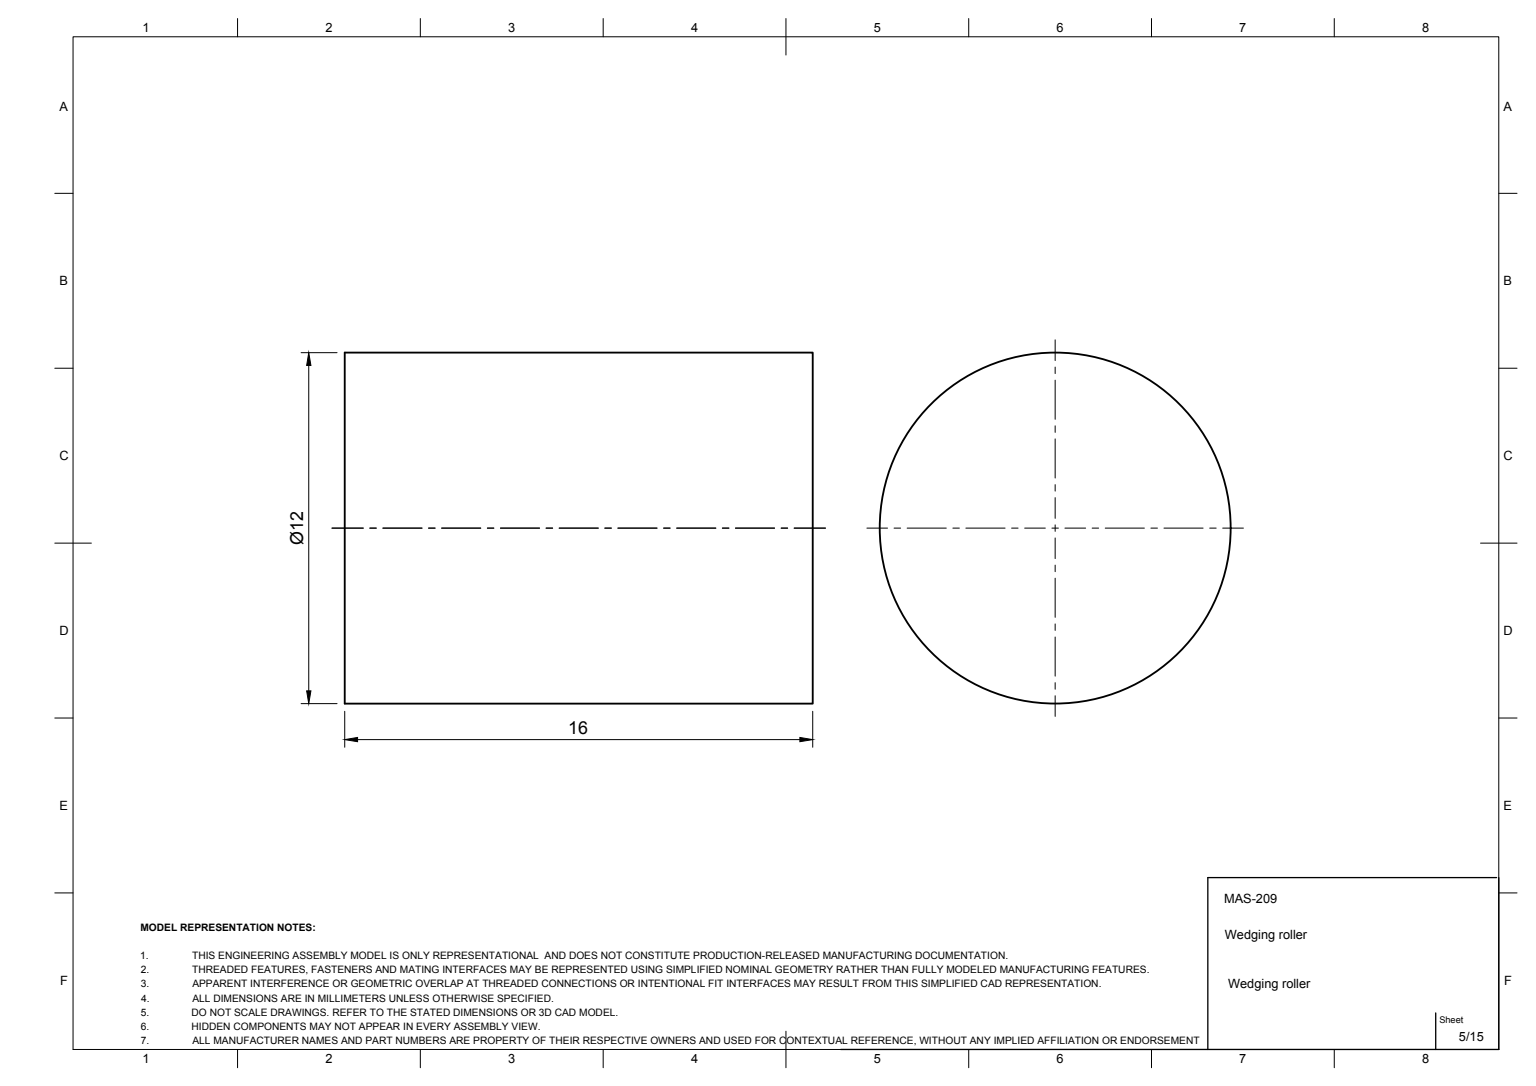
ISO-10303-21;
HEADER;
/* Generated by software containing ST-Developer
 * from STEP Tools, Inc. (www.steptools.com) 
 */

FILE_DESCRIPTION(
/* description */ ('Independent bearing-supported roller-ramp one-way clutch. Six logarit
hmic ramps with plain solid rollers, sprung guided plungers, native Co
il variants, removable shared keepers, rounded parallel key, shaft wit
h complete retaining lips, bronze journal/thrust support and bolted co
vers. Native rotor, roller planar/spin and plunger joints permit manua
l geometric engaged/released inspection. Automatic frictional torque s
witching/contact dynamics are not simulated; no capacity, hardness, fi
t, lubrication, speed, force or life rating. External input driver/cou
pling/anchors outside assembly.'),
/* implementation_level */ '2;1');

FILE_NAME(
/* name */ 'Wedging roller.step',
/* time_stamp */ '2026-11-08T07:04:38-08:00',
/* author */ (''),
/* organization */ (''),
/* preprocessor_version */ 'ST-DEVELOPER v20.2',
/* originating_system */ 'Autodesk Translation Framework v15.17.0.0',
/* authorisation */ '');

FILE_SCHEMA (('AUTOMOTIVE_DESIGN { 1 0 10303 214 3 1 1 }'));
ENDSEC;

DATA;
#10=MECHANICAL_DESIGN_GEOMETRIC_PRESENTATION_REPRESENTATION('',(#304),#99526);
#272=SHAPE_REPRESENTATION_RELATIONSHIP('SRR','None',#99629,#288);
#288=ADVANCED_BREP_SHAPE_REPRESENTATION('',(#320),#99514);
#304=STYLED_ITEM('',(#99718),#320);
#320=MANIFOLD_SOLID_BREP('Body1',#18274);
#565=PLANE('',#19493);
#566=PLANE('',#19494);
#1521=FACE_OUTER_BOUND('',#2580,.T.);
#1522=FACE_OUTER_BOUND('',#2581,.T.);
#1523=FACE_OUTER_BOUND('',#2582,.T.);
#2580=EDGE_LOOP('',(#15846,#15847,#15848,#15849));
#2581=EDGE_LOOP('',(#15850));
#2582=EDGE_LOOP('',(#15851));
#3020=CIRCLE('',#19491,6.);
#3021=CIRCLE('',#19492,6.);
#5399=LINE('',#94662,#6303);
#6303=VECTOR('',#22626,6.);
#8035=VERTEX_POINT('',#94659);
#8036=VERTEX_POINT('',#94661);
#10675=EDGE_CURVE('',#8035,#8035,#3020,.T.);
#10676=EDGE_CURVE('',#8035,#8036,#5399,.T.);
#10677=EDGE_CURVE('',#8036,#8036,#3021,.T.);
#15846=ORIENTED_EDGE('',*,*,#10675,.F.);
#15847=ORIENTED_EDGE('',*,*,#10676,.T.);
#15848=ORIENTED_EDGE('',*,*,#10677,.T.);
#15849=ORIENTED_EDGE('',*,*,#10676,.F.);
#15850=ORIENTED_EDGE('',*,*,#10675,.T.);
#15851=ORIENTED_EDGE('',*,*,#10677,.F.);
#17185=CYLINDRICAL_SURFACE('',#19490,6.);
#18119=ADVANCED_FACE('',(#1521),#17185,.T.);
#18120=ADVANCED_FACE('',(#1522),#565,.T.);
#18121=ADVANCED_FACE('',(#1523),#566,.F.);
#18274=CLOSED_SHELL('',(#18119,#18120,#18121));
#19489=AXIS2_PLACEMENT_3D('',#94657,#22620,#22621);
#19490=AXIS2_PLACEMENT_3D('',#94658,#22622,#22623);
#19491=AXIS2_PLACEMENT_3D('',#94660,#22624,#22625);
#19492=AXIS2_PLACEMENT_3D('',#94663,#22627,#22628);
#19493=AXIS2_PLACEMENT_3D('',#94664,#22629,#22630);
#19494=AXIS2_PLACEMENT_3D('',#94665,#22631,#22632);
#22620=DIRECTION('axis',(0.,0.,1.));
#22621=DIRECTION('refdir',(1.,0.,0.));
#22622=DIRECTION('center_axis',(0.,0.,1.));
#22623=DIRECTION('ref_axis',(1.,0.,0.));
#22624=DIRECTION('center_axis',(0.,0.,1.));
#22625=DIRECTION('ref_axis',(1.,0.,0.));
#22626=DIRECTION('',(0.,0.,-1.));
#22627=DIRECTION('center_axis',(0.,0.,1.));
#22628=DIRECTION('ref_axis',(1.,0.,0.));
#22629=DIRECTION('center_axis',(0.,0.,1.));
#22630=DIRECTION('ref_axis',(1.,0.,0.));
#22631=DIRECTION('center_axis',(0.,0.,1.));
#22632=DIRECTION('ref_axis',(1.,0.,0.));
#94657=CARTESIAN_POINT('',(0.,0.,0.));
#94658=CARTESIAN_POINT('Origin',(0.,0.,0.));
#94659=CARTESIAN_POINT('',(-6.,-7.34788079488412E-16,16.));
#94660=CARTESIAN_POINT('Origin',(0.,0.,16.));
#94661=CARTESIAN_POINT('',(-6.,-7.34788079488412E-16,0.));
#94662=CARTESIAN_POINT('',(-6.,-7.34788079488412E-16,0.));
#94663=CARTESIAN_POINT('Origin',(0.,0.,0.));
#94664=CARTESIAN_POINT('Origin',(0.,0.,16.));
#94665=CARTESIAN_POINT('Origin',(0.,0.,0.));
#99496=UNCERTAINTY_MEASURE_WITH_UNIT(LENGTH_MEASURE(0.01),#99527,
'DISTANCE_ACCURACY_VALUE',
'Maximum model space distance between geometric entities at asserted c
onnectivities');
#99508=UNCERTAINTY_MEASURE_WITH_UNIT(LENGTH_MEASURE(0.01),#99527,
'DISTANCE_ACCURACY_VALUE',
'Maximum model space distance between geometric entities at asserted c
onnectivities');
#99514=(
GEOMETRIC_REPRESENTATION_CONTEXT(3)
GLOBAL_UNCERTAINTY_ASSIGNED_CONTEXT((#99496))
GLOBAL_UNIT_ASSIGNED_CONTEXT((#99527,#99529,#99530))
REPRESENTATION_CONTEXT('','3D')
);
#99526=(
GEOMETRIC_REPRESENTATION_CONTEXT(3)
GLOBAL_UNCERTAINTY_ASSIGNED_CONTEXT((#99508))
GLOBAL_UNIT_ASSIGNED_CONTEXT((#99527,#99529,#99530))
REPRESENTATION_CONTEXT('','3D')
);
#99527=(
LENGTH_UNIT()
NAMED_UNIT(*)
SI_UNIT(.MILLI.,.METRE.)
);
#99529=(
NAMED_UNIT(*)
PLANE_ANGLE_UNIT()
SI_UNIT($,.RADIAN.)
);
#99530=(
NAMED_UNIT(*)
SI_UNIT($,.STERADIAN.)
SOLID_ANGLE_UNIT()
);
#99536=SHAPE_DEFINITION_REPRESENTATION(#99553,#99629);
#99553=PRODUCT_DEFINITION_SHAPE('',$,#99647);
#99629=SHAPE_REPRESENTATION('',(#19489),#99514);
#99641=PRODUCT_DEFINITION_CONTEXT('part definition',#99694,'design');
#99647=PRODUCT_DEFINITION('Wedging roller','Wedging roller',#99664,#99641);
#99664=PRODUCT_DEFINITION_FORMATION('',$,#99701);
#99694=APPLICATION_CONTEXT(
'Core Data for Automotive Mechanical Design Process');
#99695=PRODUCT_CONTEXT('part definition',#99694,'mechanical');
#99701=PRODUCT('Wedging roller','Wedging roller',$,(#99695));
#99718=PRESENTATION_STYLE_ASSIGNMENT((#99731));
#99731=SURFACE_STYLE_USAGE(.BOTH.,#99744);
#99744=SURFACE_SIDE_STYLE('',(#99757));
#99757=SURFACE_STYLE_FILL_AREA(#99770);
#99770=FILL_AREA_STYLE('Gray',(#99783));
#99783=FILL_AREA_STYLE_COLOUR('Gray',#99796);
#99796=COLOUR_RGB('Gray',0.576470588235294,0.615686274509804,0.666666666666667);
ENDSEC;
END-ISO-10303-21;
